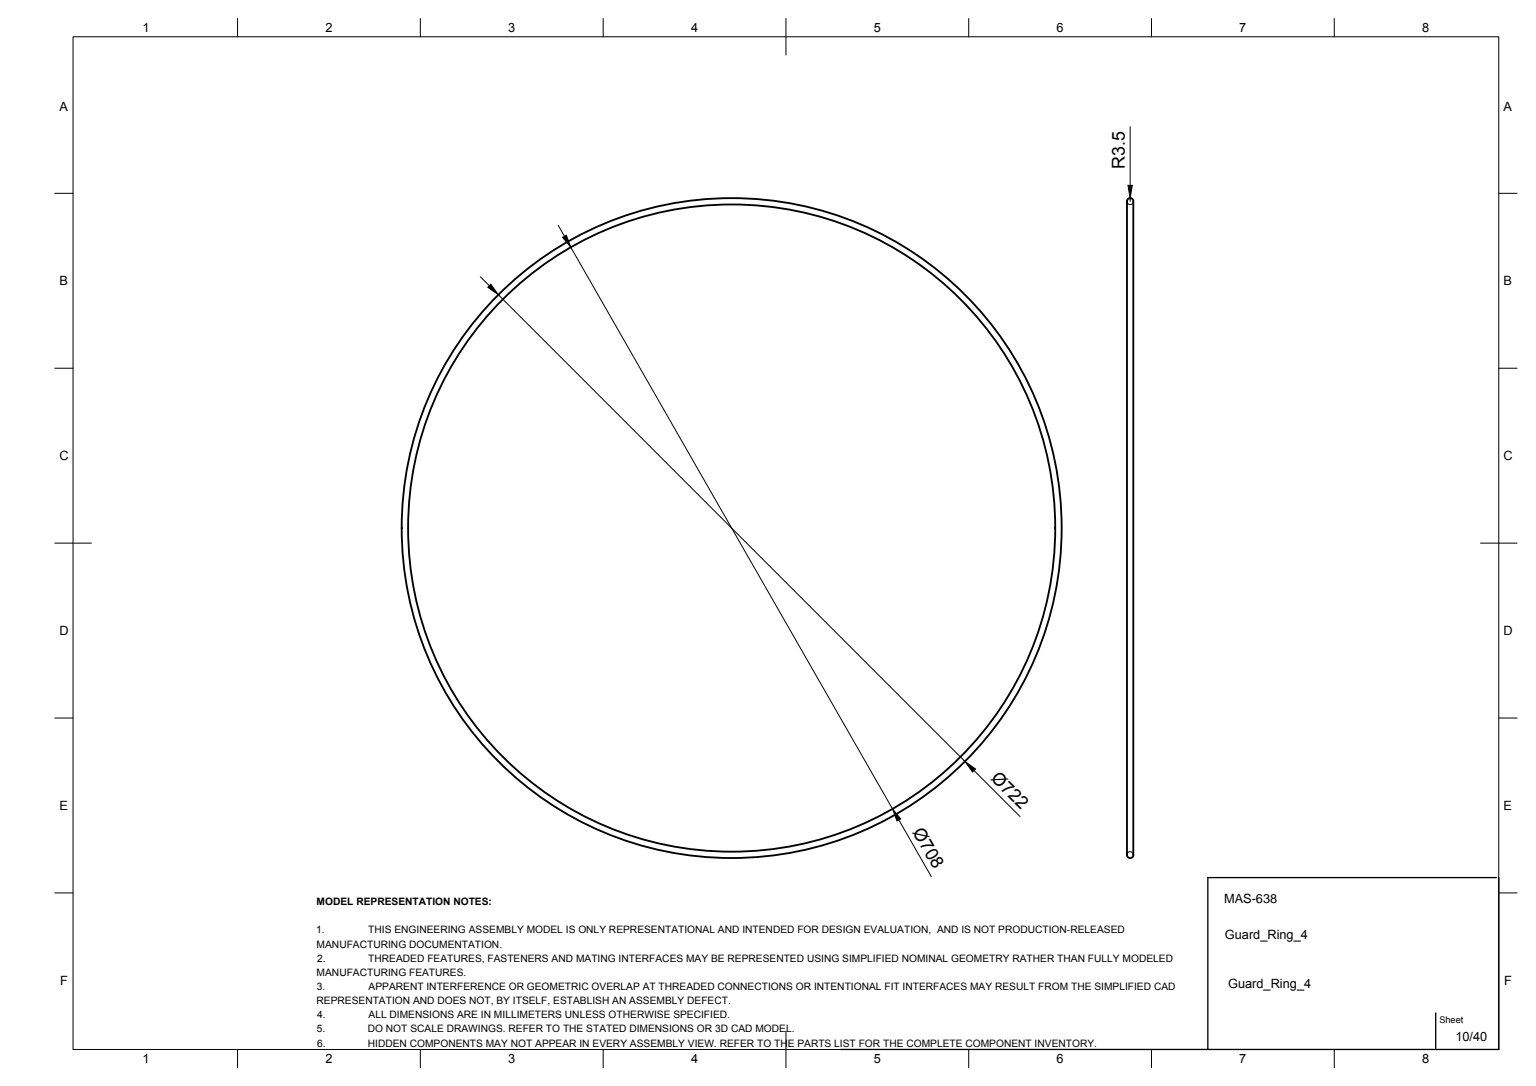
ISO-10303-21;
HEADER;
FILE_DESCRIPTION((''),'2;1');
FILE_NAME('Guard_Ring_4.step','2026-10-09T12:00:21-07:00',(''),(''),'','','');
FILE_SCHEMA (('AUTOMOTIVE_DESIGN { 1 0 10303 214 3 1 1 }'));
ENDSEC;
DATA;
#10=MECHANICAL_DESIGN_GEOMETRIC_PRESENTATION_REPRESENTATION('',(#401),#10334);
#337=SHAPE_REPRESENTATION_RELATIONSHIP('SRR','None',#10453,#369) ;
#369=ADVANCED_BREP_SHAPE_REPRESENTATION('',(#441),#10305) ;
#401=STYLED_ITEM('',(#10631),#441) ;
#441=MANIFOLD_SOLID_BREP('Body1',#3563) ;
#862=FACE_OUTER_BOUND('',#1062,.T.) ;
#1062=EDGE_LOOP('',(#2361,#2362,#2363,#2364)) ;
#1282=CIRCLE('',#3987,0.349999999999999) ;
#1283=CIRCLE('',#3988,35.4) ;
#1516=VERTEX_POINT('',#5668) ;
#1837=EDGE_CURVE('',#1516,#1516,#1282,.T.) ;
#1838=EDGE_CURVE('',#1516,#1516,#1283,.T.) ;
#2361=ORIENTED_EDGE('',*,*,#1837,.F.) ;
#2362=ORIENTED_EDGE('',*,*,#1838,.T.) ;
#2363=ORIENTED_EDGE('',*,*,#1837,.T.) ;
#2364=ORIENTED_EDGE('',*,*,#1838,.F.) ;
#3308=TOROIDAL_SURFACE('',#3986,35.75,0.349999999999999) ;
#3370=ADVANCED_FACE('',(#862),#3308,.T.) ;
#3563=CLOSED_SHELL('',(#3370)) ;
#3985=AXIS2_PLACEMENT_3D('',#5666,#4531,#4532) ;
#3986=AXIS2_PLACEMENT_3D('',#5667,#4533,#4534) ;
#3987=AXIS2_PLACEMENT_3D('',#5669,#4535,#4536) ;
#3988=AXIS2_PLACEMENT_3D('',#5670,#4537,#4538) ;
#4531=DIRECTION('axis',(0.,0.,1.)) ;
#4532=DIRECTION('refdir',(1.,0.,0.)) ;
#4533=DIRECTION('center_axis',(6.42891162084177E-17,1.,1.01883556321148E-16)) ;
#4534=DIRECTION('ref_axis',(-1.,0.,0.)) ;
#4535=DIRECTION('center_axis',(0.,1.01883556321148E-16,-1.)) ;
#4536=DIRECTION('ref_axis',(1.,0.,0.)) ;
#4537=DIRECTION('center_axis',(-6.42891162084177E-17,-1.,-1.01883556321148E-16)) ;
#4538=DIRECTION('ref_axis',(-1.,6.42891162084177E-17,6.55000379205715E-33)) ;
#5666=CARTESIAN_POINT('',(0.,0.,0.)) ;
#5667=CARTESIAN_POINT('Origin',(23.47768801576,64.5830586252741,68.2224337400009)) ;
#5668=CARTESIAN_POINT('',(58.87768801576,64.5830586252741,68.2224337400009)) ;
#5669=CARTESIAN_POINT('Origin',(59.22768801576,64.5830586252741,68.2224337400009)) ;
#5670=CARTESIAN_POINT('Origin',(23.47768801576,64.5830586252741,68.2224337400009)) ;
#10268=UNCERTAINTY_MEASURE_WITH_UNIT(LENGTH_MEASURE(0.001),#10335,
'DISTANCE_ACCURACY_VALUE',
'Maximum model space distance between geometric entities at asserted c
onnectivities') ;
#10297=UNCERTAINTY_MEASURE_WITH_UNIT(LENGTH_MEASURE(0.001),#10335,
'DISTANCE_ACCURACY_VALUE',
'Maximum model space distance between geometric entities at asserted c
onnectivities') ;
#10305=(
GEOMETRIC_REPRESENTATION_CONTEXT(3)
GLOBAL_UNCERTAINTY_ASSIGNED_CONTEXT((#10268))
GLOBAL_UNIT_ASSIGNED_CONTEXT((#10335,#10337,#10338))
REPRESENTATION_CONTEXT('','3D')
) ;
#10334=(
GEOMETRIC_REPRESENTATION_CONTEXT(3)
GLOBAL_UNCERTAINTY_ASSIGNED_CONTEXT((#10297))
GLOBAL_UNIT_ASSIGNED_CONTEXT((#10335,#10337,#10338))
REPRESENTATION_CONTEXT('','3D')
) ;
#10335=(
LENGTH_UNIT()
NAMED_UNIT(*)
SI_UNIT(.CENTI.,.METRE.)
) ;
#10337=(
NAMED_UNIT(*)
PLANE_ANGLE_UNIT()
SI_UNIT($,.RADIAN.)
) ;
#10338=(
NAMED_UNIT(*)
SI_UNIT($,.STERADIAN.)
SOLID_ANGLE_UNIT()
) ;
#10346=SHAPE_DEFINITION_REPRESENTATION(#10382,#10453) ;
#10382=PRODUCT_DEFINITION_SHAPE('',$,#10490) ;
#10453=SHAPE_REPRESENTATION('',(#3985),#10305) ;
#10482=PRODUCT_DEFINITION_CONTEXT('part definition',#10592,'design') ;
#10490=PRODUCT_DEFINITION('Guard_Ring_4','Guard_Ring_4',#10526,#10482) ;
#10526=PRODUCT_DEFINITION_FORMATION('',$,#10601) ;
#10592=APPLICATION_CONTEXT(
'Core Data for Automotive Mechanical Design Process') ;
#10593=PRODUCT_CONTEXT('part definition',#10592,'mechanical') ;
#10601=PRODUCT('Guard_Ring_4','Guard_Ring_4',$,(#10593)) ;
#10631=PRESENTATION_STYLE_ASSIGNMENT((#10635)) ;
#10635=SURFACE_STYLE_USAGE(.BOTH.,#10639) ;
#10639=SURFACE_SIDE_STYLE('',(#10643)) ;
#10643=SURFACE_STYLE_FILL_AREA(#10647) ;
#10647=FILL_AREA_STYLE('Opaque(25,25,25)',(#10651)) ;
#10651=FILL_AREA_STYLE_COLOUR('Opaque(25,25,25)',#10655) ;
#10655=COLOUR_RGB('Opaque(25,25,25)', 0.09019608, 0.27058824, 0.51372549) ;
ENDSEC;
END-ISO-10303-21;
